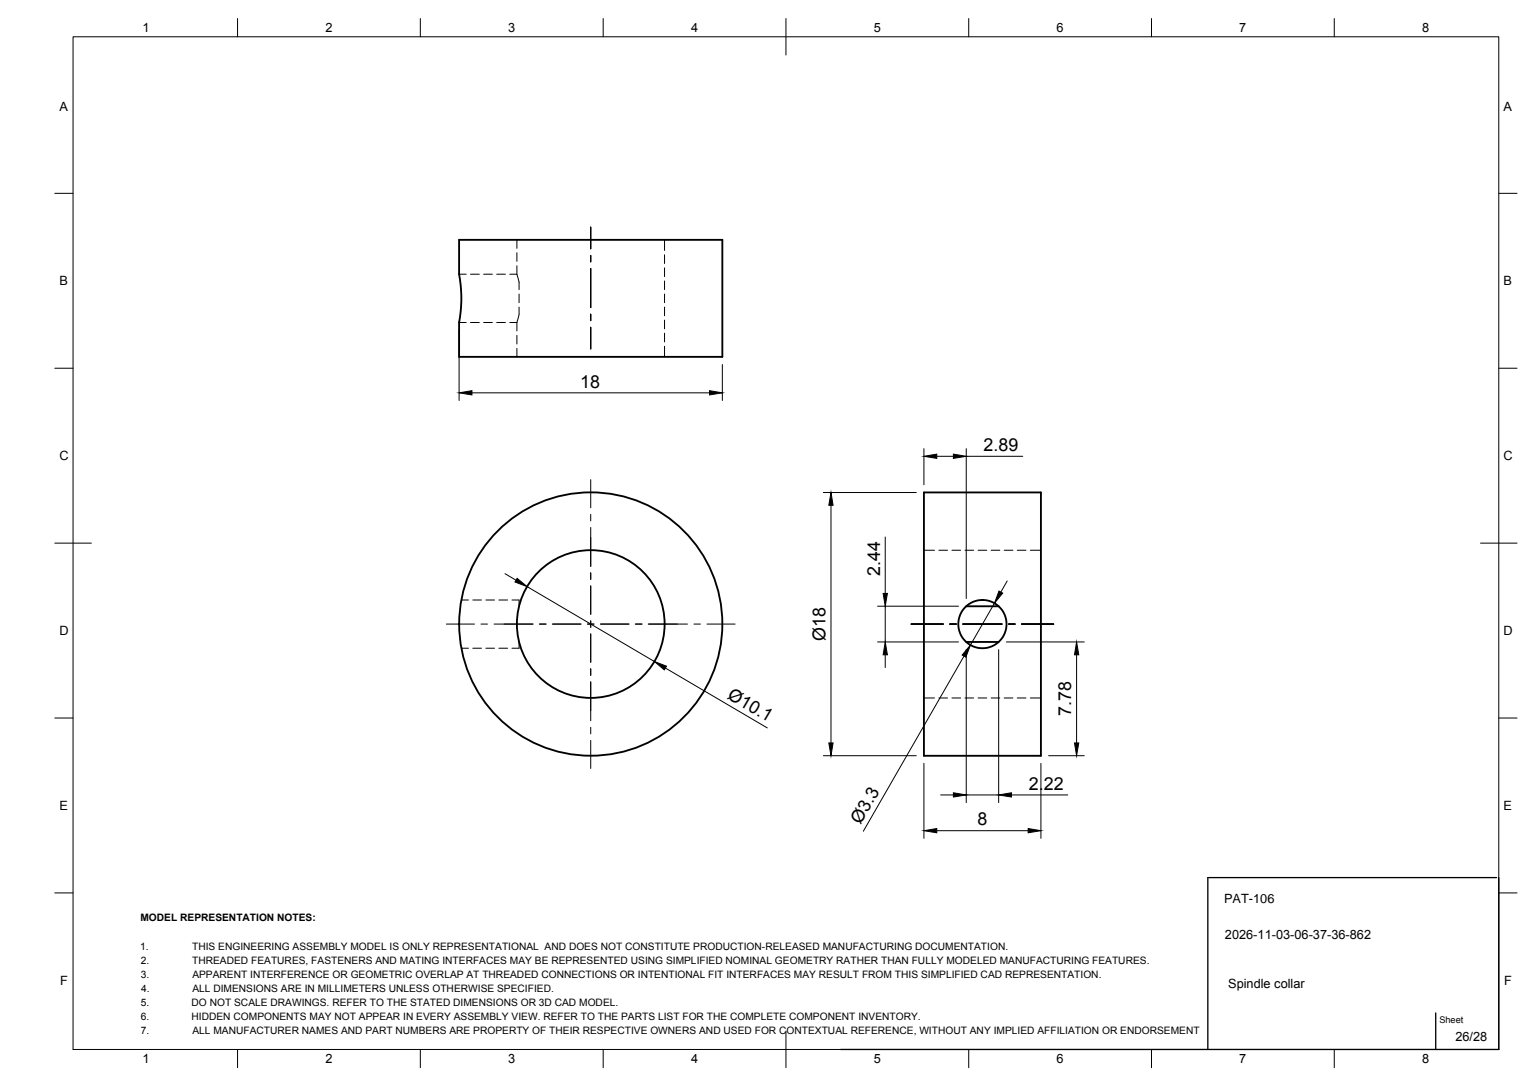
ISO-10303-21;
HEADER;
/* Generated by software containing ST-Developer
 * from STEP Tools, Inc. (www.steptools.com) 
 */

FILE_DESCRIPTION(
/* description */ ('Torsion-spring ratchet demonstrator'),
/* implementation_level */ '2;1');

FILE_NAME(
/* name */ 'Spindle collar.step',
/* time_stamp */ '2026-10-29T17:29:17-07:00',
/* author */ (''),
/* organization */ (''),
/* preprocessor_version */ 'ST-DEVELOPER v20.2',
/* originating_system */ 'Autodesk Translation Framework v15.17.0.0',
/* authorisation */ '');

FILE_SCHEMA (('AUTOMOTIVE_DESIGN { 1 0 10303 214 3 1 1 }'));
ENDSEC;

DATA;
#10=MECHANICAL_DESIGN_GEOMETRIC_PRESENTATION_REPRESENTATION('',(#310),#11258);
#226=B_SPLINE_CURVE_WITH_KNOTS('',3,(#10535,#10536,#10537,#10538,#10539,
#10540,#10541,#10542,#10543,#10544,#10545,#10546,#10547,#10548),
 .UNSPECIFIED.,.F.,.F.,(4,2,2,2,2,2,4),(0.618551524396293,0.626563103102765,
0.689203386094988,0.751843669087211,0.814483952079434,0.877124235071657,
0.88513581377813),.UNSPECIFIED.);
#227=B_SPLINE_CURVE_WITH_KNOTS('',3,(#10552,#10553,#10554,#10555,#10556,
#10557,#10558,#10559),.UNSPECIFIED.,.F.,.F.,(4,2,2,4),(0.250614556362404,
0.313254839354627,0.37589512234685,0.383906701053323),.UNSPECIFIED.);
#228=B_SPLINE_CURVE_WITH_KNOTS('',3,(#10563,#10564,#10565,#10566,#10567,
#10568,#10569,#10570,#10571,#10572,#10573,#10574,#10575,#10576,#10577,#10578,
#10579,#10580,#10581,#10582,#10583,#10584,#10585,#10586,#10587,#10588),
 .UNSPECIFIED.,.F.,.F.,(4,2,2,2,2,2,2,2,2,2,2,2,4),(0.,0.0623062782223143,
0.124612556444629,0.186916384615149,0.249220212785669,0.31152404095619,
0.37382786912671,0.436134147349024,0.498440425571339,0.560746703793653,
0.623052982015967,0.685356810186488,0.747660638357008),.UNSPECIFIED.);
#229=B_SPLINE_CURVE_WITH_KNOTS('',3,(#10589,#10590,#10591,#10592,#10593,
#10594,#10595,#10596,#10597,#10598),.UNSPECIFIED.,.F.,.F.,(4,2,2,2,4),(0.747660638357008,
0.809964466527528,0.872268294698049,0.934574572920363,0.996880851142677),
 .UNSPECIFIED.);
#230=B_SPLINE_CURVE_WITH_KNOTS('',3,(#10599,#10600,#10601,#10602,#10603,
#10604,#10605,#10606),.UNSPECIFIED.,.F.,.F.,(4,2,2,4),(0.117322411671485,
0.125333990377958,0.187974273370181,0.250614556362404),.UNSPECIFIED.);
#254=SHAPE_REPRESENTATION_RELATIONSHIP('SRR','None',#11382,#278);
#278=ADVANCED_BREP_SHAPE_REPRESENTATION('',(#340),#11252);
#310=STYLED_ITEM('',(#11577),#340);
#340=MANIFOLD_SOLID_BREP('Body1',#5183);
#424=FACE_BOUND('',#1214,.T.);
#425=FACE_BOUND('',#1216,.T.);
#426=FACE_BOUND('',#1218,.T.);
#427=FACE_BOUND('',#1220,.T.);
#536=PLANE('',#5919);
#537=PLANE('',#5923);
#538=PLANE('',#5930);
#539=PLANE('',#5931);
#826=FACE_OUTER_BOUND('',#1210,.T.);
#827=FACE_OUTER_BOUND('',#1211,.T.);
#828=FACE_OUTER_BOUND('',#1212,.T.);
#829=FACE_OUTER_BOUND('',#1213,.T.);
#830=FACE_OUTER_BOUND('',#1215,.T.);
#831=FACE_OUTER_BOUND('',#1217,.T.);
#832=FACE_OUTER_BOUND('',#1219,.T.);
#1210=EDGE_LOOP('',(#4242,#4243));
#1211=EDGE_LOOP('',(#4244,#4245,#4246,#4247,#4248,#4249,#4250,#4251,#4252));
#1212=EDGE_LOOP('',(#4253,#4254));
#1213=EDGE_LOOP('',(#4255,#4256,#4257,#4258));
#1214=EDGE_LOOP('',(#4259,#4260,#4261,#4262,#4263));
#1215=EDGE_LOOP('',(#4264,#4265,#4266,#4267));
#1216=EDGE_LOOP('',(#4268,#4269));
#1217=EDGE_LOOP('',(#4270));
#1218=EDGE_LOOP('',(#4271));
#1219=EDGE_LOOP('',(#4272));
#1220=EDGE_LOOP('',(#4273));
#1486=LINE('',#10531,#1869);
#1487=LINE('',#10561,#1870);
#1488=LINE('',#10608,#1871);
#1489=LINE('',#10613,#1872);
#1490=LINE('',#10619,#1873);
#1869=VECTOR('',#7161,1.);
#1870=VECTOR('',#7168,0.165);
#1871=VECTOR('',#7171,1.);
#1872=VECTOR('',#7176,0.505);
#1873=VECTOR('',#7183,0.9);
#2305=CIRCLE('',#5920,0.165);
#2306=CIRCLE('',#5922,0.165);
#2307=CIRCLE('',#5925,0.505);
#2308=CIRCLE('',#5926,0.505);
#2309=CIRCLE('',#5928,0.9);
#2310=CIRCLE('',#5929,0.9);
#2609=VERTEX_POINT('',#10529);
#2610=VERTEX_POINT('',#10530);
#2611=VERTEX_POINT('',#10534);
#2612=VERTEX_POINT('',#10549);
#2613=VERTEX_POINT('',#10551);
#2614=VERTEX_POINT('',#10560);
#2615=VERTEX_POINT('',#10562);
#2616=VERTEX_POINT('',#10610);
#2617=VERTEX_POINT('',#10612);
#2618=VERTEX_POINT('',#10616);
#2619=VERTEX_POINT('',#10618);
#3181=EDGE_CURVE('',#2609,#2610,#1486,.T.);
#3182=EDGE_CURVE('',#2609,#2610,#2305,.T.);
#3183=EDGE_CURVE('',#2611,#2609,#226,.T.);
#3184=EDGE_CURVE('',#2612,#2611,#2306,.T.);
#3185=EDGE_CURVE('',#2613,#2612,#227,.T.);
#3186=EDGE_CURVE('',#2613,#2614,#1487,.T.);
#3187=EDGE_CURVE('',#2615,#2614,#228,.T.);
#3188=EDGE_CURVE('',#2614,#2615,#229,.T.);
#3189=EDGE_CURVE('',#2610,#2613,#230,.T.);
#3190=EDGE_CURVE('',#2612,#2611,#1488,.T.);
#3191=EDGE_CURVE('',#2616,#2616,#2307,.T.);
#3192=EDGE_CURVE('',#2616,#2617,#1489,.T.);
#3193=EDGE_CURVE('',#2617,#2617,#2308,.T.);
#3194=EDGE_CURVE('',#2618,#2618,#2309,.T.);
#3195=EDGE_CURVE('',#2618,#2619,#1490,.T.);
#3196=EDGE_CURVE('',#2619,#2619,#2310,.T.);
#4242=ORIENTED_EDGE('',*,*,#3181,.F.);
#4243=ORIENTED_EDGE('',*,*,#3182,.T.);
#4244=ORIENTED_EDGE('',*,*,#3183,.F.);
#4245=ORIENTED_EDGE('',*,*,#3184,.F.);
#4246=ORIENTED_EDGE('',*,*,#3185,.F.);
#4247=ORIENTED_EDGE('',*,*,#3186,.T.);
#4248=ORIENTED_EDGE('',*,*,#3187,.F.);
#4249=ORIENTED_EDGE('',*,*,#3188,.F.);
#4250=ORIENTED_EDGE('',*,*,#3186,.F.);
#4251=ORIENTED_EDGE('',*,*,#3189,.F.);
#4252=ORIENTED_EDGE('',*,*,#3182,.F.);
#4253=ORIENTED_EDGE('',*,*,#3190,.F.);
#4254=ORIENTED_EDGE('',*,*,#3184,.T.);
#4255=ORIENTED_EDGE('',*,*,#3191,.F.);
#4256=ORIENTED_EDGE('',*,*,#3192,.T.);
#4257=ORIENTED_EDGE('',*,*,#3193,.T.);
#4258=ORIENTED_EDGE('',*,*,#3192,.F.);
#4259=ORIENTED_EDGE('',*,*,#3189,.T.);
#4260=ORIENTED_EDGE('',*,*,#3185,.T.);
#4261=ORIENTED_EDGE('',*,*,#3190,.T.);
#4262=ORIENTED_EDGE('',*,*,#3183,.T.);
#4263=ORIENTED_EDGE('',*,*,#3181,.T.);
#4264=ORIENTED_EDGE('',*,*,#3194,.F.);
#4265=ORIENTED_EDGE('',*,*,#3195,.T.);
#4266=ORIENTED_EDGE('',*,*,#3196,.T.);
#4267=ORIENTED_EDGE('',*,*,#3195,.F.);
#4268=ORIENTED_EDGE('',*,*,#3187,.T.);
#4269=ORIENTED_EDGE('',*,*,#3188,.T.);
#4270=ORIENTED_EDGE('',*,*,#3194,.T.);
#4271=ORIENTED_EDGE('',*,*,#3191,.T.);
#4272=ORIENTED_EDGE('',*,*,#3196,.F.);
#4273=ORIENTED_EDGE('',*,*,#3193,.F.);
#4837=CYLINDRICAL_SURFACE('',#5921,0.165);
#4838=CYLINDRICAL_SURFACE('',#5924,0.505);
#4839=CYLINDRICAL_SURFACE('',#5927,0.9);
#5052=ADVANCED_FACE('',(#826),#536,.T.);
#5053=ADVANCED_FACE('',(#827),#4837,.F.);
#5054=ADVANCED_FACE('',(#828),#537,.T.);
#5055=ADVANCED_FACE('',(#829,#424),#4838,.F.);
#5056=ADVANCED_FACE('',(#830,#425),#4839,.T.);
#5057=ADVANCED_FACE('',(#831,#426),#538,.T.);
#5058=ADVANCED_FACE('',(#832,#427),#539,.F.);
#5183=CLOSED_SHELL('',(#5052,#5053,#5054,#5055,#5056,#5057,#5058));
#5918=AXIS2_PLACEMENT_3D('',#10527,#7157,#7158);
#5919=AXIS2_PLACEMENT_3D('',#10528,#7159,#7160);
#5920=AXIS2_PLACEMENT_3D('',#10532,#7162,#7163);
#5921=AXIS2_PLACEMENT_3D('',#10533,#7164,#7165);
#5922=AXIS2_PLACEMENT_3D('',#10550,#7166,#7167);
#5923=AXIS2_PLACEMENT_3D('',#10607,#7169,#7170);
#5924=AXIS2_PLACEMENT_3D('',#10609,#7172,#7173);
#5925=AXIS2_PLACEMENT_3D('',#10611,#7174,#7175);
#5926=AXIS2_PLACEMENT_3D('',#10614,#7177,#7178);
#5927=AXIS2_PLACEMENT_3D('',#10615,#7179,#7180);
#5928=AXIS2_PLACEMENT_3D('',#10617,#7181,#7182);
#5929=AXIS2_PLACEMENT_3D('',#10620,#7184,#7185);
#5930=AXIS2_PLACEMENT_3D('',#10621,#7186,#7187);
#5931=AXIS2_PLACEMENT_3D('',#10622,#7188,#7189);
#7157=DIRECTION('axis',(0.,0.,1.));
#7158=DIRECTION('refdir',(1.,0.,0.));
#7159=DIRECTION('center_axis',(1.,0.,0.));
#7160=DIRECTION('ref_axis',(0.,0.,-1.));
#7161=DIRECTION('',(0.,0.,1.));
#7162=DIRECTION('center_axis',(1.,0.,0.));
#7163=DIRECTION('ref_axis',(0.,0.,-1.));
#7164=DIRECTION('center_axis',(1.,0.,0.));
#7165=DIRECTION('ref_axis',(0.,0.,-1.));
#7166=DIRECTION('center_axis',(1.,0.,0.));
#7167=DIRECTION('ref_axis',(0.,0.,-1.));
#7168=DIRECTION('',(1.,0.,0.));
#7169=DIRECTION('center_axis',(1.,0.,0.));
#7170=DIRECTION('ref_axis',(0.,0.,-1.));
#7171=DIRECTION('',(0.,0.,-1.));
#7172=DIRECTION('center_axis',(0.,0.,1.));
#7173=DIRECTION('ref_axis',(1.,0.,0.));
#7174=DIRECTION('center_axis',(0.,0.,-1.));
#7175=DIRECTION('ref_axis',(1.,0.,0.));
#7176=DIRECTION('',(0.,0.,-1.));
#7177=DIRECTION('center_axis',(0.,0.,-1.));
#7178=DIRECTION('ref_axis',(1.,0.,0.));
#7179=DIRECTION('center_axis',(0.,0.,1.));
#7180=DIRECTION('ref_axis',(1.,0.,0.));
#7181=DIRECTION('center_axis',(0.,0.,1.));
#7182=DIRECTION('ref_axis',(1.,0.,0.));
#7183=DIRECTION('',(0.,0.,-1.));
#7184=DIRECTION('center_axis',(0.,0.,1.));
#7185=DIRECTION('ref_axis',(1.,0.,0.));
#7186=DIRECTION('center_axis',(0.,0.,1.));
#7187=DIRECTION('ref_axis',(1.,0.,0.));
#7188=DIRECTION('center_axis',(0.,0.,1.));
#7189=DIRECTION('ref_axis',(1.,0.,0.));
#10527=CARTESIAN_POINT('',(0.,0.,0.));
#10528=CARTESIAN_POINT('Origin',(0.49,0.,1.4));
#10529=CARTESIAN_POINT('',(0.49,0.122167917228706,1.28909463493591));
#10530=CARTESIAN_POINT('',(0.49,0.122167917228706,1.51090536506409));
#10531=CARTESIAN_POINT('',(0.49,0.122167917228706,1.));
#10532=CARTESIAN_POINT('Origin',(0.49,0.,1.4));
#10533=CARTESIAN_POINT('Origin',(0.49,0.,1.4));
#10534=CARTESIAN_POINT('',(0.49,-0.122167917228706,1.28909463493591));
#10535=CARTESIAN_POINT('Ctrl Pts',(0.49,-0.122167917228706,1.28909463493591));
#10536=CARTESIAN_POINT('Ctrl Pts',(0.490448531679987,-0.120368913626296,
1.28711294069536));
#10537=CARTESIAN_POINT('Ctrl Pts',(0.490895245371685,-0.118534896565231,
1.28518965877367));
#10538=CARTESIAN_POINT('Ctrl Pts',(0.494795015531646,-0.102111993019358,
1.2687667552278));
#10539=CARTESIAN_POINT('Ctrl Pts',(0.498442514607594,-0.0836597150224318,
1.25609154388858));
#10540=CARTESIAN_POINT('Ctrl Pts',(0.50357781976106,-0.0430495960471595,
1.23920409039234));
#10541=CARTESIAN_POINT('Ctrl Pts',(0.505,-0.020880094330741,1.235));
#10542=CARTESIAN_POINT('Ctrl Pts',(0.505,0.020880094330741,1.235));
#10543=CARTESIAN_POINT('Ctrl Pts',(0.50357781976106,0.0430495960471595,
1.23920409039234));
#10544=CARTESIAN_POINT('Ctrl Pts',(0.498442514607594,0.0836597150224318,
1.25609154388858));
#10545=CARTESIAN_POINT('Ctrl Pts',(0.494795015531646,0.102111993019358,
1.2687667552278));
#10546=CARTESIAN_POINT('Ctrl Pts',(0.490895245371684,0.118534896565231,
1.28518965877367));
#10547=CARTESIAN_POINT('Ctrl Pts',(0.490448531679987,0.120368913626296,
1.28711294069536));
#10548=CARTESIAN_POINT('Ctrl Pts',(0.49,0.122167917228706,1.28909463493591));
#10549=CARTESIAN_POINT('',(0.49,-0.122167917228706,1.51090536506409));
#10550=CARTESIAN_POINT('Origin',(0.49,0.,1.4));
#10551=CARTESIAN_POINT('',(0.505,-1.70422299968729E-17,1.565));
#10552=CARTESIAN_POINT('Ctrl Pts',(0.505,-6.93889390390723E-18,1.565));
#10553=CARTESIAN_POINT('Ctrl Pts',(0.505,-0.020880094330741,1.565));
#10554=CARTESIAN_POINT('Ctrl Pts',(0.50357781976106,-0.0430495960471595,
1.56079590960766));
#10555=CARTESIAN_POINT('Ctrl Pts',(0.498442514607594,-0.0836597150224318,
1.54390845611142));
#10556=CARTESIAN_POINT('Ctrl Pts',(0.494795015531646,-0.102111993019358,
1.5312332447722));
#10557=CARTESIAN_POINT('Ctrl Pts',(0.490895245371684,-0.118534896565231,
1.51481034122633));
#10558=CARTESIAN_POINT('Ctrl Pts',(0.490448531679987,-0.120368913626296,
1.51288705930464));
#10559=CARTESIAN_POINT('Ctrl Pts',(0.49,-0.122167917228706,1.51090536506409));
#10560=CARTESIAN_POINT('',(0.9,-2.02066721859313E-17,1.565));
#10561=CARTESIAN_POINT('',(0.49,-2.02066721859313E-17,1.565));
#10562=CARTESIAN_POINT('',(0.884745726183518,0.165,1.4));
#10563=CARTESIAN_POINT('Ctrl Pts',(0.884745726183518,0.165,1.4));
#10564=CARTESIAN_POINT('Ctrl Pts',(0.884745726183518,0.165,1.37923124059256));
#10565=CARTESIAN_POINT('Ctrl Pts',(0.885552759505264,0.160839719007584,
1.35711110492666));
#10566=CARTESIAN_POINT('Ctrl Pts',(0.888448648150043,0.143986470216691,
1.31647293736623));
#10567=CARTESIAN_POINT('Ctrl Pts',(0.890493604851638,0.131295993814186,
1.29795075602263));
#10568=CARTESIAN_POINT('Ctrl Pts',(0.89431723432394,0.102049819008125,1.26870458121656));
#10569=CARTESIAN_POINT('Ctrl Pts',(0.896347088899543,0.0835273920906824,
1.25601365401642));
#10570=CARTESIAN_POINT('Ctrl Pts',(0.899208271860583,0.0428883760934127,
1.23916007816136));
#10571=CARTESIAN_POINT('Ctrl Pts',(0.9,0.0207679427235068,1.235));
#10572=CARTESIAN_POINT('Ctrl Pts',(0.9,-0.0207679427235068,1.235));
#10573=CARTESIAN_POINT('Ctrl Pts',(0.899208271860583,-0.0428883760934127,
1.23916007816136));
#10574=CARTESIAN_POINT('Ctrl Pts',(0.896347088899543,-0.0835273920906823,
1.25601365401642));
#10575=CARTESIAN_POINT('Ctrl Pts',(0.89431723432394,-0.102049819008125,
1.26870458121656));
#10576=CARTESIAN_POINT('Ctrl Pts',(0.890493604851638,-0.131295993814186,
1.29795075602263));
#10577=CARTESIAN_POINT('Ctrl Pts',(0.888448648150043,-0.143986470216691,
1.31647293736623));
#10578=CARTESIAN_POINT('Ctrl Pts',(0.885552759505264,-0.160839719007584,
1.35711110492666));
#10579=CARTESIAN_POINT('Ctrl Pts',(0.884745726183518,-0.165,1.37923124059256));
#10580=CARTESIAN_POINT('Ctrl Pts',(0.884745726183518,-0.165,1.42076875940744));
#10581=CARTESIAN_POINT('Ctrl Pts',(0.885552759505264,-0.160839719007584,
1.44288889507334));
#10582=CARTESIAN_POINT('Ctrl Pts',(0.888448648150043,-0.14398647021669,
1.48352706263377));
#10583=CARTESIAN_POINT('Ctrl Pts',(0.890493604851638,-0.131295993814186,
1.50204924397737));
#10584=CARTESIAN_POINT('Ctrl Pts',(0.89431723432394,-0.102049819008125,
1.53129541878344));
#10585=CARTESIAN_POINT('Ctrl Pts',(0.896347088899543,-0.0835273920906824,
1.54398634598358));
#10586=CARTESIAN_POINT('Ctrl Pts',(0.899208271860583,-0.0428883760934128,
1.56083992183864));
#10587=CARTESIAN_POINT('Ctrl Pts',(0.9,-0.0207679427235068,1.565));
#10588=CARTESIAN_POINT('Ctrl Pts',(0.9,-6.93889390390723E-18,1.565));
#10589=CARTESIAN_POINT('Ctrl Pts',(0.9,-3.46944695195361E-17,1.565));
#10590=CARTESIAN_POINT('Ctrl Pts',(0.9,0.0207679427235068,1.565));
#10591=CARTESIAN_POINT('Ctrl Pts',(0.899208271860583,0.0428883760934127,
1.56083992183864));
#10592=CARTESIAN_POINT('Ctrl Pts',(0.896347088899543,0.0835273920906824,
1.54398634598358));
#10593=CARTESIAN_POINT('Ctrl Pts',(0.89431723432394,0.102049819008125,1.53129541878344));
#10594=CARTESIAN_POINT('Ctrl Pts',(0.890493604851638,0.131295993814186,
1.50204924397737));
#10595=CARTESIAN_POINT('Ctrl Pts',(0.888448648150043,0.143986470216691,
1.48352706263377));
#10596=CARTESIAN_POINT('Ctrl Pts',(0.885552759505264,0.160839719007584,
1.44288889507334));
#10597=CARTESIAN_POINT('Ctrl Pts',(0.884745726183518,0.165,1.42076875940744));
#10598=CARTESIAN_POINT('Ctrl Pts',(0.884745726183518,0.165,1.4));
#10599=CARTESIAN_POINT('Ctrl Pts',(0.49,0.122167917228706,1.51090536506409));
#10600=CARTESIAN_POINT('Ctrl Pts',(0.490448531679987,0.120368913626296,
1.51288705930464));
#10601=CARTESIAN_POINT('Ctrl Pts',(0.490895245371685,0.118534896565231,
1.51481034122633));
#10602=CARTESIAN_POINT('Ctrl Pts',(0.494795015531646,0.102111993019358,
1.5312332447722));
#10603=CARTESIAN_POINT('Ctrl Pts',(0.498442514607594,0.0836597150224318,
1.54390845611142));
#10604=CARTESIAN_POINT('Ctrl Pts',(0.50357781976106,0.0430495960471594,
1.56079590960766));
#10605=CARTESIAN_POINT('Ctrl Pts',(0.505,0.020880094330741,1.565));
#10606=CARTESIAN_POINT('Ctrl Pts',(0.505,0.,1.565));
#10607=CARTESIAN_POINT('Origin',(0.49,0.,1.4));
#10608=CARTESIAN_POINT('',(0.49,-0.122167917228706,1.));
#10609=CARTESIAN_POINT('Origin',(0.,0.,1.));
#10610=CARTESIAN_POINT('',(-0.505,-6.18446633569413E-17,1.8));
#10611=CARTESIAN_POINT('Origin',(0.,0.,1.8));
#10612=CARTESIAN_POINT('',(-0.505,-6.18446633569413E-17,1.));
#10613=CARTESIAN_POINT('',(-0.505,-6.18446633569413E-17,1.));
#10614=CARTESIAN_POINT('Origin',(0.,0.,1.));
#10615=CARTESIAN_POINT('Origin',(0.,0.,1.));
#10616=CARTESIAN_POINT('',(-0.9,-1.10218211923262E-16,1.8));
#10617=CARTESIAN_POINT('Origin',(0.,0.,1.8));
#10618=CARTESIAN_POINT('',(-0.9,-1.10218211923262E-16,1.));
#10619=CARTESIAN_POINT('',(-0.9,-1.10218211923262E-16,1.));
#10620=CARTESIAN_POINT('Origin',(0.,0.,1.));
#10621=CARTESIAN_POINT('Origin',(0.,0.,1.8));
#10622=CARTESIAN_POINT('Origin',(0.,0.,1.));
#11222=UNCERTAINTY_MEASURE_WITH_UNIT(LENGTH_MEASURE(0.001),#11259,
'DISTANCE_ACCURACY_VALUE',
'Maximum model space distance between geometric entities at asserted c
onnectivities');
#11228=UNCERTAINTY_MEASURE_WITH_UNIT(LENGTH_MEASURE(0.001),#11259,
'DISTANCE_ACCURACY_VALUE',
'Maximum model space distance between geometric entities at asserted c
onnectivities');
#11252=(
GEOMETRIC_REPRESENTATION_CONTEXT(3)
GLOBAL_UNCERTAINTY_ASSIGNED_CONTEXT((#11222))
GLOBAL_UNIT_ASSIGNED_CONTEXT((#11259,#11261,#11262))
REPRESENTATION_CONTEXT('','3D')
);
#11258=(
GEOMETRIC_REPRESENTATION_CONTEXT(3)
GLOBAL_UNCERTAINTY_ASSIGNED_CONTEXT((#11228))
GLOBAL_UNIT_ASSIGNED_CONTEXT((#11259,#11261,#11262))
REPRESENTATION_CONTEXT('','3D')
);
#11259=(
LENGTH_UNIT()
NAMED_UNIT(*)
SI_UNIT(.CENTI.,.METRE.)
);
#11261=(
NAMED_UNIT(*)
PLANE_ANGLE_UNIT()
SI_UNIT($,.RADIAN.)
);
#11262=(
NAMED_UNIT(*)
SI_UNIT($,.STERADIAN.)
SOLID_ANGLE_UNIT()
);
#11286=SHAPE_DEFINITION_REPRESENTATION(#11343,#11382);
#11343=PRODUCT_DEFINITION_SHAPE('',$,#11412);
#11382=SHAPE_REPRESENTATION('',(#5918),#11252);
#11388=PRODUCT_DEFINITION_CONTEXT('part definition',#11477,'design');
#11412=PRODUCT_DEFINITION('Spindle collar','Spindle collar',#11441,#11388);
#11441=PRODUCT_DEFINITION_FORMATION('',$,#11502);
#11477=APPLICATION_CONTEXT(
'Core Data for Automotive Mechanical Design Process');
#11478=PRODUCT_CONTEXT('part definition',#11477,'mechanical');
#11502=PRODUCT('Spindle collar','Spindle collar','Spindle collar',(#11478));
#11571=COLOUR_RGB('Sky Blue',0.24,0.69,0.87);
#11572=FILL_AREA_STYLE_COLOUR('',#11571);
#11573=FILL_AREA_STYLE('',(#11572));
#11574=SURFACE_STYLE_FILL_AREA(#11573);
#11575=SURFACE_SIDE_STYLE('',(#11574));
#11576=SURFACE_STYLE_USAGE(.BOTH.,#11575);
#11577=PRESENTATION_STYLE_ASSIGNMENT((#11576));
ENDSEC;
END-ISO-10303-21;
